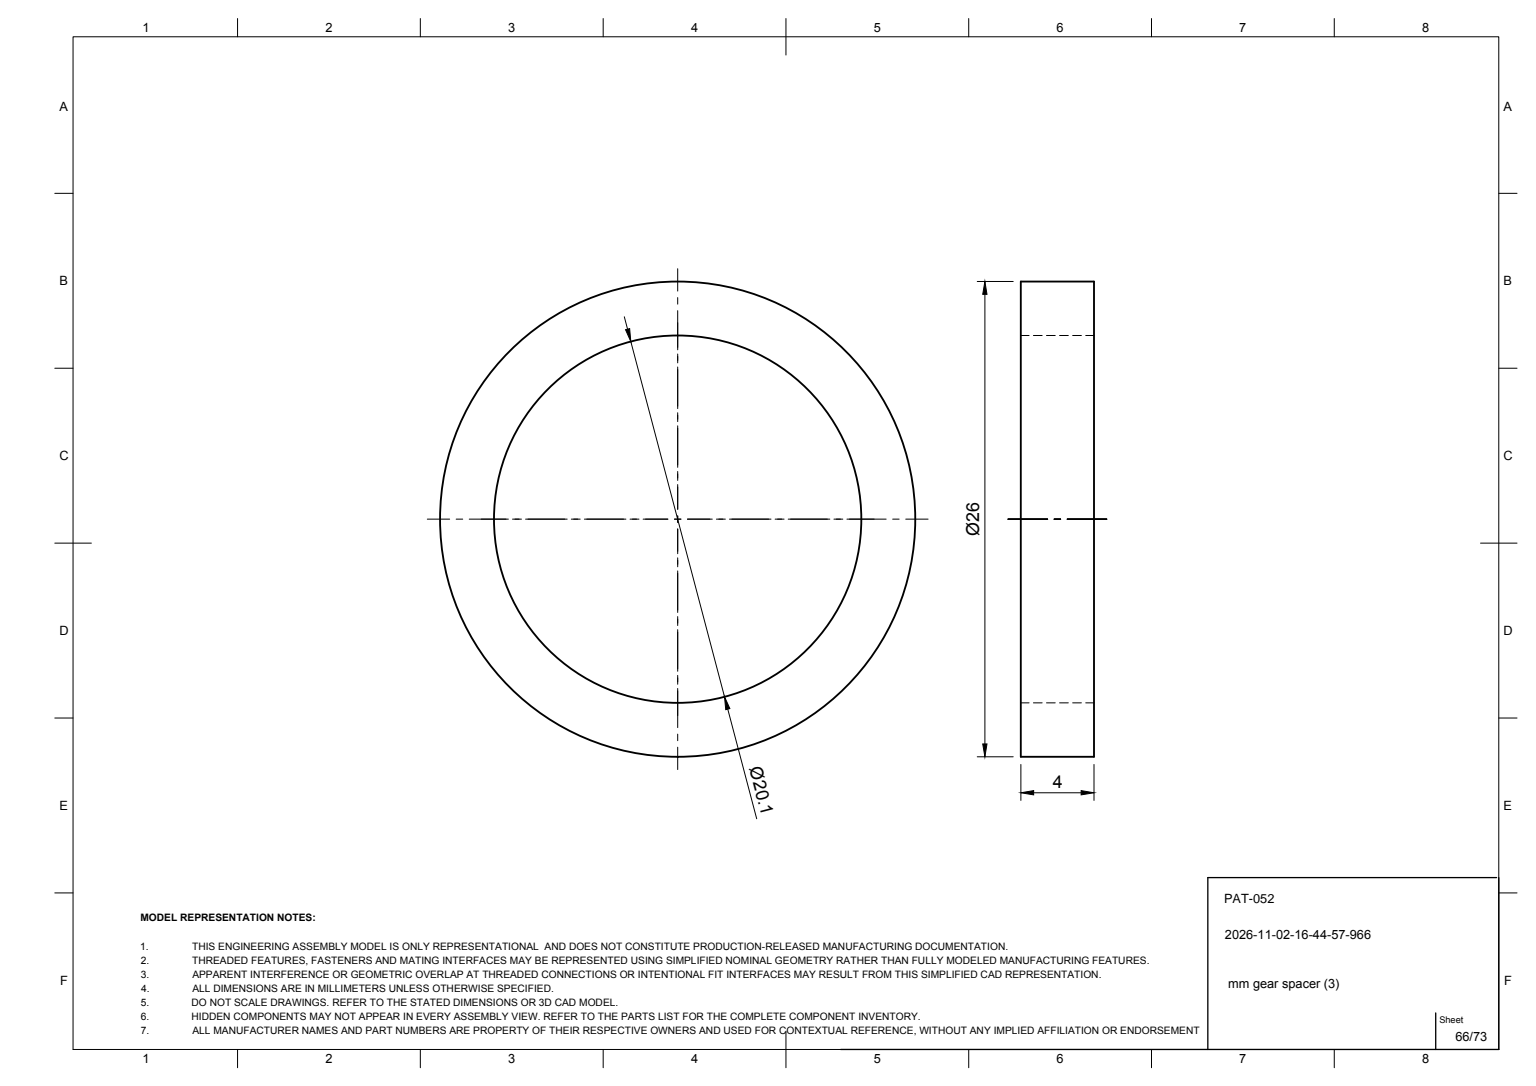
ISO-10303-21;
HEADER;
/* Generated by software containing ST-Developer
 * from STEP Tools, Inc. (www.steptools.com) 
 */

FILE_DESCRIPTION(
/* description */ ('Hand-crank gear train demonstrator'),
/* implementation_level */ '2;1');

FILE_NAME(
/* name */ 'mm gear spacer (3).step',
/* time_stamp */ '2026-10-28T03:22:13-07:00',
/* author */ (''),
/* organization */ (''),
/* preprocessor_version */ 'ST-DEVELOPER v20.2',
/* originating_system */ 'Autodesk Translation Framework v15.17.0.0',
/* authorisation */ '');

FILE_SCHEMA (('AUTOMOTIVE_DESIGN { 1 0 10303 214 3 1 1 }'));
ENDSEC;

DATA;
#10=MECHANICAL_DESIGN_GEOMETRIC_PRESENTATION_REPRESENTATION('',(#1256),#62758);
#1113=SHAPE_REPRESENTATION_RELATIONSHIP('SRR','None',#63091,#1177);
#1177=ADVANCED_BREP_SHAPE_REPRESENTATION('',(#1331),#62745);
#1256=STYLED_ITEM('',(#63476),#1331);
#1331=MANIFOLD_SOLID_BREP('Body1',#16440);
#1607=FACE_BOUND('',#4014,.T.);
#1608=FACE_BOUND('',#4016,.T.);
#2023=PLANE('',#18408);
#2024=PLANE('',#18409);
#2810=FACE_OUTER_BOUND('',#4011,.T.);
#2811=FACE_OUTER_BOUND('',#4012,.T.);
#2812=FACE_OUTER_BOUND('',#4013,.T.);
#2813=FACE_OUTER_BOUND('',#4015,.T.);
#4011=EDGE_LOOP('',(#13861,#13862,#13863,#13864));
#4012=EDGE_LOOP('',(#13865,#13866,#13867,#13868));
#4013=EDGE_LOOP('',(#13869));
#4014=EDGE_LOOP('',(#13870));
#4015=EDGE_LOOP('',(#13871));
#4016=EDGE_LOOP('',(#13872));
#5149=LINE('',#38483,#6281);
#5150=LINE('',#38489,#6282);
#6281=VECTOR('',#22186,1.005);
#6282=VECTOR('',#22193,1.3);
#7076=CIRCLE('',#18403,1.005);
#7077=CIRCLE('',#18404,1.005);
#7078=CIRCLE('',#18406,1.3);
#7079=CIRCLE('',#18407,1.3);
#8235=VERTEX_POINT('',#38480);
#8236=VERTEX_POINT('',#38482);
#8237=VERTEX_POINT('',#38486);
#8238=VERTEX_POINT('',#38488);
#10182=EDGE_CURVE('',#8235,#8235,#7076,.T.);
#10183=EDGE_CURVE('',#8235,#8236,#5149,.T.);
#10184=EDGE_CURVE('',#8236,#8236,#7077,.T.);
#10185=EDGE_CURVE('',#8237,#8237,#7078,.T.);
#10186=EDGE_CURVE('',#8237,#8238,#5150,.T.);
#10187=EDGE_CURVE('',#8238,#8238,#7079,.T.);
#13861=ORIENTED_EDGE('',*,*,#10182,.F.);
#13862=ORIENTED_EDGE('',*,*,#10183,.T.);
#13863=ORIENTED_EDGE('',*,*,#10184,.T.);
#13864=ORIENTED_EDGE('',*,*,#10183,.F.);
#13865=ORIENTED_EDGE('',*,*,#10185,.F.);
#13866=ORIENTED_EDGE('',*,*,#10186,.T.);
#13867=ORIENTED_EDGE('',*,*,#10187,.T.);
#13868=ORIENTED_EDGE('',*,*,#10186,.F.);
#13869=ORIENTED_EDGE('',*,*,#10185,.T.);
#13870=ORIENTED_EDGE('',*,*,#10182,.T.);
#13871=ORIENTED_EDGE('',*,*,#10187,.F.);
#13872=ORIENTED_EDGE('',*,*,#10184,.F.);
#15370=CYLINDRICAL_SURFACE('',#18402,1.005);
#15371=CYLINDRICAL_SURFACE('',#18405,1.3);
#16120=ADVANCED_FACE('',(#2810),#15370,.F.);
#16121=ADVANCED_FACE('',(#2811),#15371,.T.);
#16122=ADVANCED_FACE('',(#2812,#1607),#2023,.T.);
#16123=ADVANCED_FACE('',(#2813,#1608),#2024,.F.);
#16440=CLOSED_SHELL('',(#16120,#16121,#16122,#16123));
#18401=AXIS2_PLACEMENT_3D('',#38478,#22180,#22181);
#18402=AXIS2_PLACEMENT_3D('',#38479,#22182,#22183);
#18403=AXIS2_PLACEMENT_3D('',#38481,#22184,#22185);
#18404=AXIS2_PLACEMENT_3D('',#38484,#22187,#22188);
#18405=AXIS2_PLACEMENT_3D('',#38485,#22189,#22190);
#18406=AXIS2_PLACEMENT_3D('',#38487,#22191,#22192);
#18407=AXIS2_PLACEMENT_3D('',#38490,#22194,#22195);
#18408=AXIS2_PLACEMENT_3D('',#38491,#22196,#22197);
#18409=AXIS2_PLACEMENT_3D('',#38492,#22198,#22199);
#22180=DIRECTION('axis',(0.,0.,1.));
#22181=DIRECTION('refdir',(1.,0.,0.));
#22182=DIRECTION('center_axis',(0.,1.,0.));
#22183=DIRECTION('ref_axis',(1.,0.,0.));
#22184=DIRECTION('center_axis',(0.,-1.,0.));
#22185=DIRECTION('ref_axis',(1.,0.,0.));
#22186=DIRECTION('',(0.,-1.,0.));
#22187=DIRECTION('center_axis',(0.,-1.,0.));
#22188=DIRECTION('ref_axis',(1.,0.,0.));
#22189=DIRECTION('center_axis',(0.,1.,0.));
#22190=DIRECTION('ref_axis',(1.,0.,0.));
#22191=DIRECTION('center_axis',(0.,1.,0.));
#22192=DIRECTION('ref_axis',(1.,0.,0.));
#22193=DIRECTION('',(0.,-1.,0.));
#22194=DIRECTION('center_axis',(0.,1.,0.));
#22195=DIRECTION('ref_axis',(1.,0.,0.));
#22196=DIRECTION('center_axis',(0.,1.,0.));
#22197=DIRECTION('ref_axis',(1.,0.,0.));
#22198=DIRECTION('center_axis',(0.,1.,0.));
#22199=DIRECTION('ref_axis',(1.,0.,0.));
#38478=CARTESIAN_POINT('',(0.,0.,0.));
#38479=CARTESIAN_POINT('Origin',(18.,-0.4,9.));
#38480=CARTESIAN_POINT('',(16.995,0.,9.));
#38481=CARTESIAN_POINT('Origin',(18.,0.,9.));
#38482=CARTESIAN_POINT('',(16.995,-0.4,9.));
#38483=CARTESIAN_POINT('',(16.995,-0.4,9.));
#38484=CARTESIAN_POINT('Origin',(18.,-0.4,9.));
#38485=CARTESIAN_POINT('Origin',(18.,-0.4,9.));
#38486=CARTESIAN_POINT('',(16.7,0.,9.));
#38487=CARTESIAN_POINT('Origin',(18.,0.,9.));
#38488=CARTESIAN_POINT('',(16.7,-0.4,9.));
#38489=CARTESIAN_POINT('',(16.7,-0.4,9.));
#38490=CARTESIAN_POINT('Origin',(18.,-0.4,9.));
#38491=CARTESIAN_POINT('Origin',(18.,0.,9.));
#38492=CARTESIAN_POINT('Origin',(18.,-0.4,9.));
#62671=UNCERTAINTY_MEASURE_WITH_UNIT(LENGTH_MEASURE(0.001),#62759,
'DISTANCE_ACCURACY_VALUE',
'Maximum model space distance between geometric entities at asserted c
onnectivities');
#62684=UNCERTAINTY_MEASURE_WITH_UNIT(LENGTH_MEASURE(0.001),#62759,
'DISTANCE_ACCURACY_VALUE',
'Maximum model space distance between geometric entities at asserted c
onnectivities');
#62745=(
GEOMETRIC_REPRESENTATION_CONTEXT(3)
GLOBAL_UNCERTAINTY_ASSIGNED_CONTEXT((#62671))
GLOBAL_UNIT_ASSIGNED_CONTEXT((#62759,#62761,#62762))
REPRESENTATION_CONTEXT('','3D')
);
#62758=(
GEOMETRIC_REPRESENTATION_CONTEXT(3)
GLOBAL_UNCERTAINTY_ASSIGNED_CONTEXT((#62684))
GLOBAL_UNIT_ASSIGNED_CONTEXT((#62759,#62761,#62762))
REPRESENTATION_CONTEXT('','3D')
);
#62759=(
LENGTH_UNIT()
NAMED_UNIT(*)
SI_UNIT(.CENTI.,.METRE.)
);
#62761=(
NAMED_UNIT(*)
PLANE_ANGLE_UNIT()
SI_UNIT($,.RADIAN.)
);
#62762=(
NAMED_UNIT(*)
SI_UNIT($,.STERADIAN.)
SOLID_ANGLE_UNIT()
);
#62823=SHAPE_DEFINITION_REPRESENTATION(#62906,#63091);
#62906=PRODUCT_DEFINITION_SHAPE('',$,#63165);
#63091=SHAPE_REPRESENTATION('',(#18401),#62745);
#63104=PRODUCT_DEFINITION_CONTEXT('part definition',#63325,'design');
#63165=PRODUCT_DEFINITION('mm gear spacer (3)','mm gear spacer (3)',#63238,
#63104);
#63238=PRODUCT_DEFINITION_FORMATION('',$,#63387);
#63325=APPLICATION_CONTEXT(
'Core Data for Automotive Mechanical Design Process');
#63326=PRODUCT_CONTEXT('part definition',#63325,'mechanical');
#63387=PRODUCT('mm gear spacer (3)','mm gear spacer (3)','mm gear spacer (3)',
(#63326));
#63470=COLOUR_RGB('Off White',0.89,0.88,0.83);
#63471=FILL_AREA_STYLE_COLOUR('',#63470);
#63472=FILL_AREA_STYLE('',(#63471));
#63473=SURFACE_STYLE_FILL_AREA(#63472);
#63474=SURFACE_SIDE_STYLE('',(#63473));
#63475=SURFACE_STYLE_USAGE(.BOTH.,#63474);
#63476=PRESENTATION_STYLE_ASSIGNMENT((#63475));
ENDSEC;
END-ISO-10303-21;
